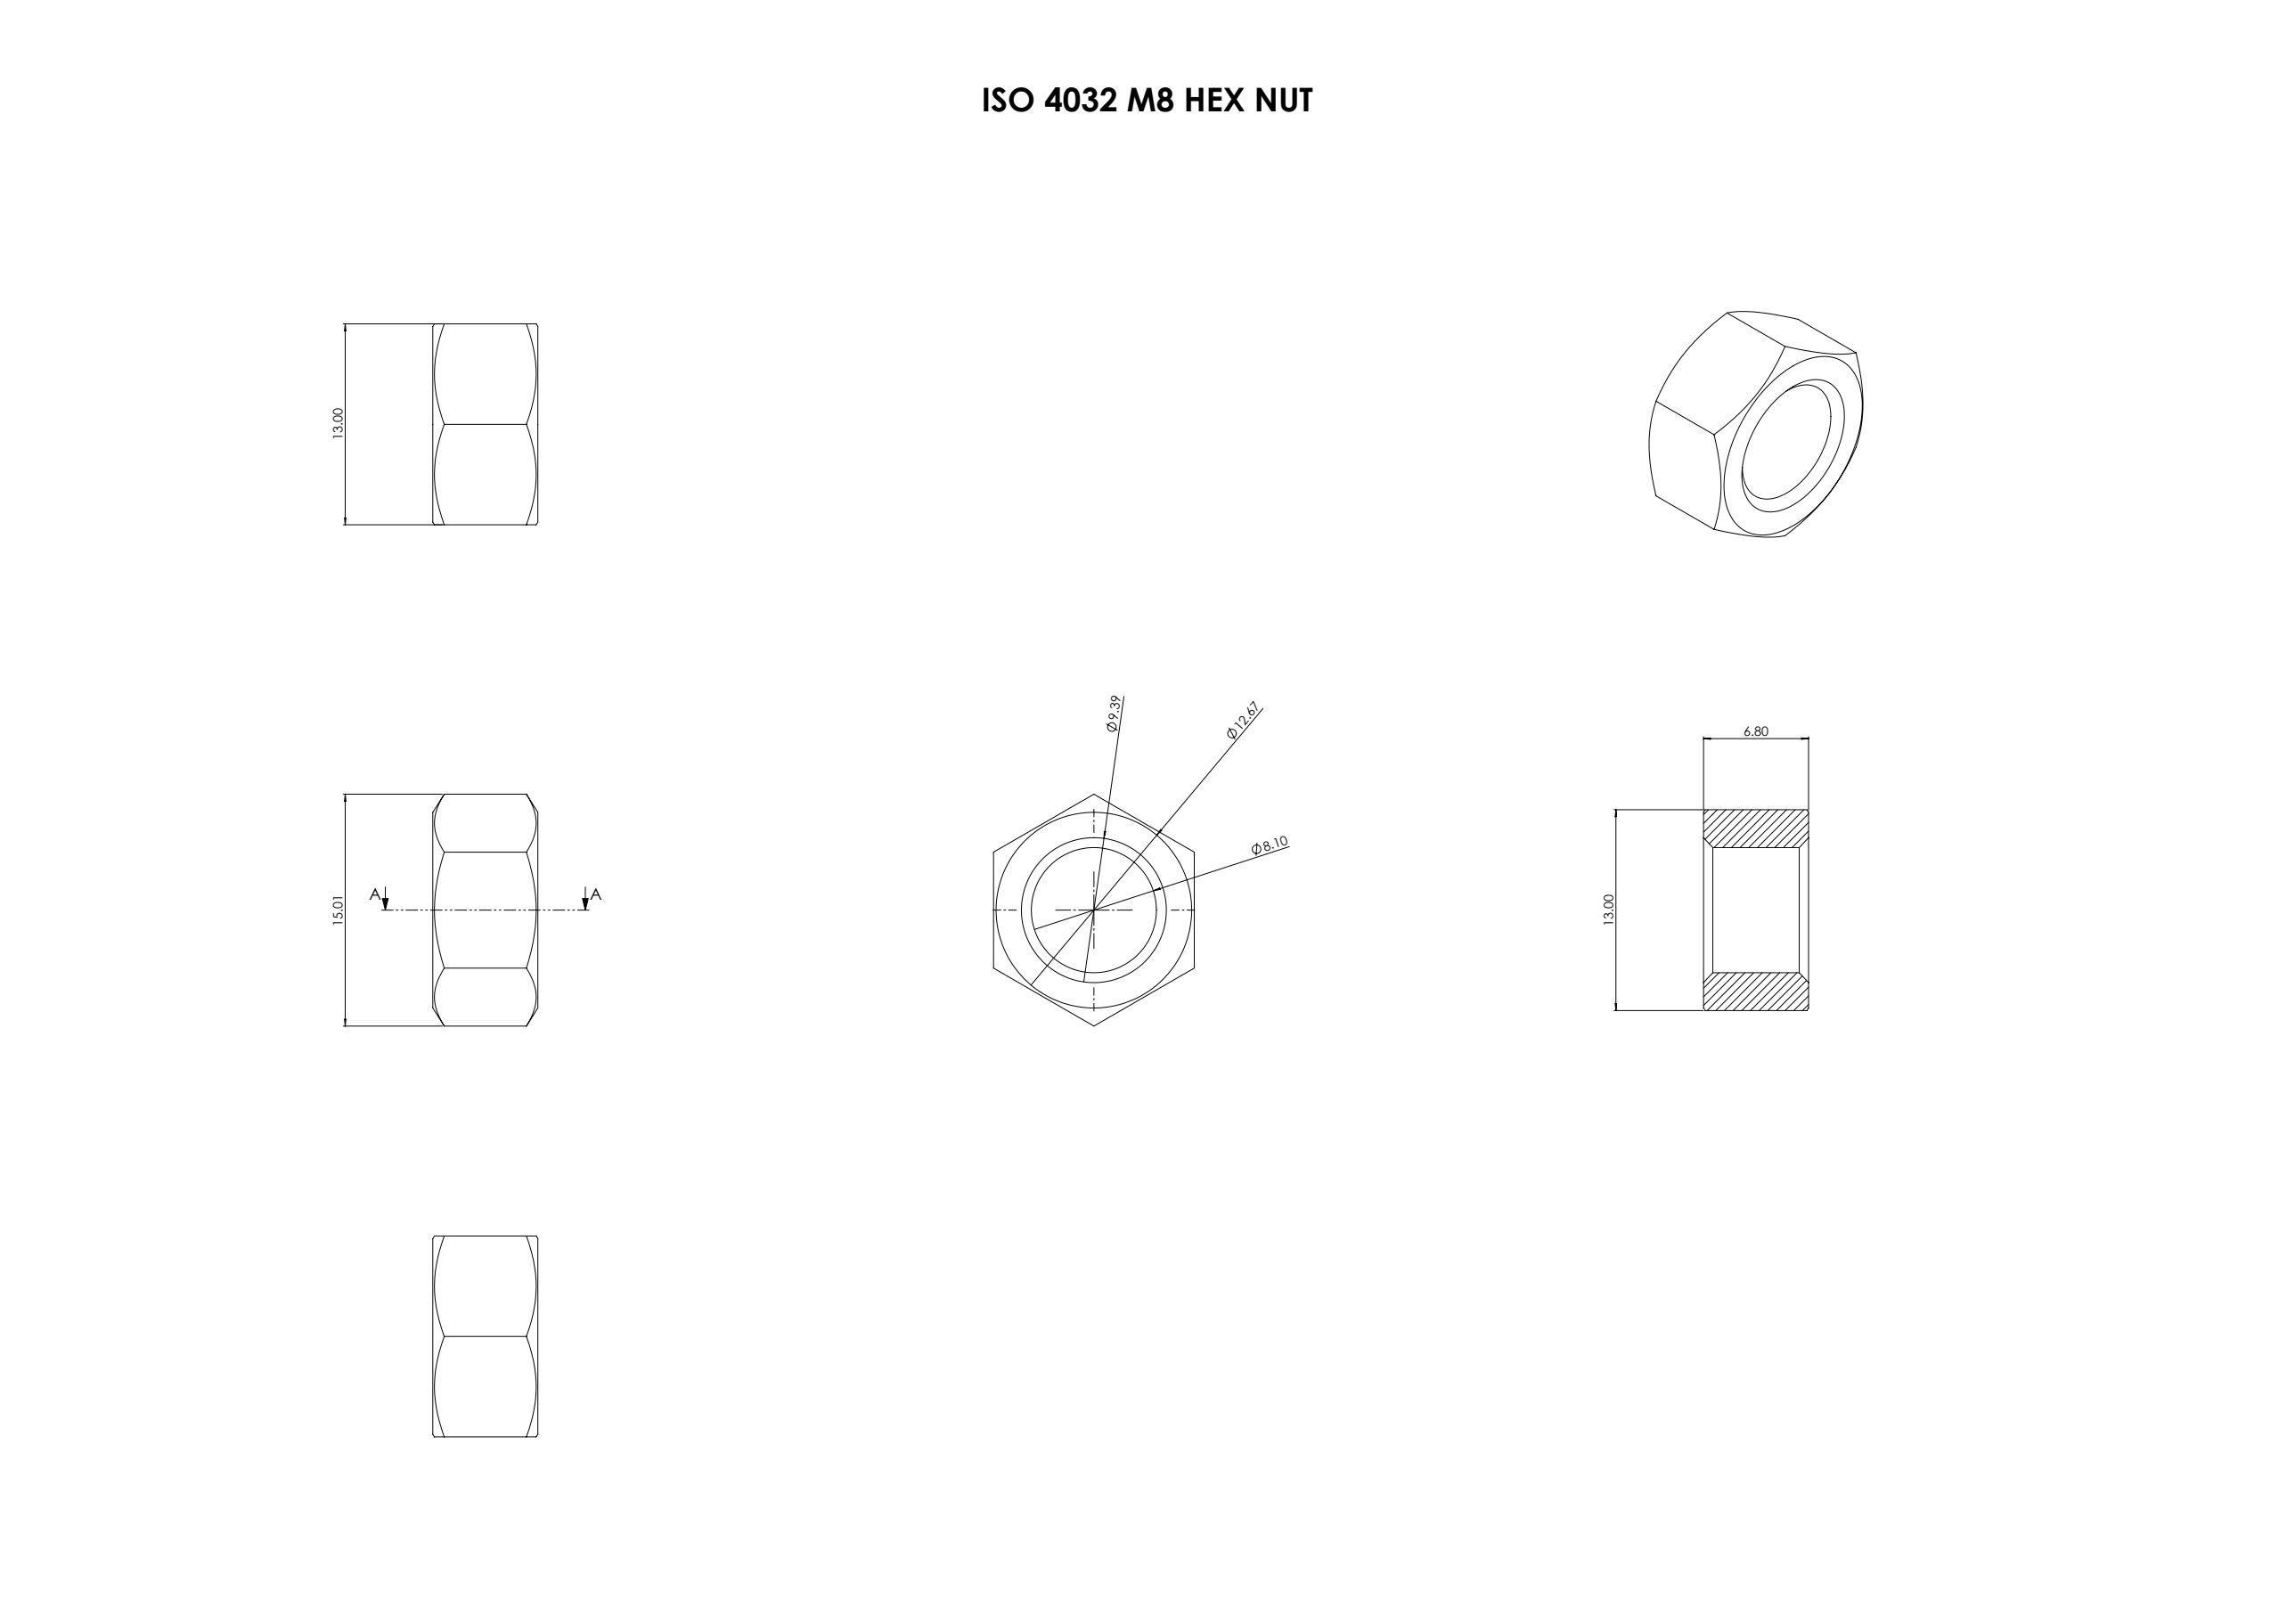
ISO-10303-21;
HEADER;
/* Generated by software containing ST-Developer
 * from STEP Tools, Inc. (www.steptools.com) 
 */

FILE_DESCRIPTION(
/* description */ (''),
/* implementation_level */ '2;1');

FILE_NAME(
/* name */ '14_ISO_4032_M8_Hex_Nut.step',
/* time_stamp */ '2026-10-11T08:27:52-07:00',
/* author */ (''),
/* organization */ (''),
/* preprocessor_version */ 'ST-DEVELOPER v20.2',
/* originating_system */ 'Autodesk Translation Framework v15.15.0.0',
/* authorisation */ '');

FILE_SCHEMA (('AUTOMOTIVE_DESIGN { 1 0 10303 214 3 1 1 }'));
ENDSEC;

DATA;
#10=MECHANICAL_DESIGN_GEOMETRIC_PRESENTATION_REPRESENTATION('',(#932),#94301);
#904=SHAPE_REPRESENTATION_RELATIONSHIP('SRR','None',#94384,#918);
#918=ADVANCED_BREP_SHAPE_REPRESENTATION('',(#946),#94300);
#932=STYLED_ITEM('',(#94588),#946);
#946=MANIFOLD_SOLID_BREP('Body1',#51031);
#1042=FACE_BOUND('',#18695,.T.);
#1043=FACE_BOUND('',#18697,.T.);
#1287=CYLINDRICAL_SURFACE('',#55318,4.05);
#6677=LINE('',#94156,#11205);
#6678=LINE('',#94160,#11206);
#6679=LINE('',#94164,#11207);
#6680=LINE('',#94170,#11208);
#6681=LINE('',#94196,#11209);
#6682=LINE('',#94201,#11210);
#6683=LINE('',#94204,#11211);
#6684=LINE('',#94210,#11212);
#6685=LINE('',#94224,#11213);
#6686=LINE('',#94230,#11214);
#6687=LINE('',#94232,#11215);
#11205=VECTOR('',#68145,4.425);
#11206=VECTOR('',#68150,4.05);
#11207=VECTOR('',#68155,4.425);
#11208=VECTOR('',#68162,7.09027674973257);
#11209=VECTOR('',#68165,10.);
#11210=VECTOR('',#68166,10.);
#11211=VECTOR('',#68169,10.);
#11212=VECTOR('',#68172,10.);
#11213=VECTOR('',#68175,7.09027674973257);
#11214=VECTOR('',#68180,10.);
#11215=VECTOR('',#68183,10.);
#13241=PLANE('',#55324);
#13242=PLANE('',#55325);
#13243=PLANE('',#55326);
#13244=PLANE('',#55329);
#13245=PLANE('',#55330);
#13246=PLANE('',#55331);
#13247=PLANE('',#55332);
#13248=PLANE('',#55333);
#15918=FACE_OUTER_BOUND('',#18683,.T.);
#15919=FACE_OUTER_BOUND('',#18684,.T.);
#15920=FACE_OUTER_BOUND('',#18685,.T.);
#15921=FACE_OUTER_BOUND('',#18686,.T.);
#15922=FACE_OUTER_BOUND('',#18687,.T.);
#15923=FACE_OUTER_BOUND('',#18688,.T.);
#15924=FACE_OUTER_BOUND('',#18689,.T.);
#15925=FACE_OUTER_BOUND('',#18690,.T.);
#15926=FACE_OUTER_BOUND('',#18691,.T.);
#15927=FACE_OUTER_BOUND('',#18692,.T.);
#15928=FACE_OUTER_BOUND('',#18693,.T.);
#15929=FACE_OUTER_BOUND('',#18694,.T.);
#15930=FACE_OUTER_BOUND('',#18696,.T.);
#18683=EDGE_LOOP('',(#48057,#48058,#48059,#48060));
#18684=EDGE_LOOP('',(#48061,#48062,#48063,#48064));
#18685=EDGE_LOOP('',(#48065,#48066,#48067,#48068));
#18686=EDGE_LOOP('',(#48069,#48070,#48071,#48072,#48073,#48074,#48075,#48076,
#48077));
#18687=EDGE_LOOP('',(#48078,#48079,#48080,#48081));
#18688=EDGE_LOOP('',(#48082,#48083,#48084,#48085));
#18689=EDGE_LOOP('',(#48086,#48087,#48088,#48089));
#18690=EDGE_LOOP('',(#48090,#48091,#48092,#48093,#48094,#48095,#48096,#48097,
#48098));
#18691=EDGE_LOOP('',(#48099,#48100,#48101,#48102));
#18692=EDGE_LOOP('',(#48103,#48104,#48105,#48106));
#18693=EDGE_LOOP('',(#48107,#48108,#48109,#48110));
#18694=EDGE_LOOP('',(#48111));
#18695=EDGE_LOOP('',(#48112));
#18696=EDGE_LOOP('',(#48113));
#18697=EDGE_LOOP('',(#48114));
#19562=(
BOUNDED_CURVE()
B_SPLINE_CURVE(2,(#94172,#94173,#94174),.UNSPECIFIED.,.F.,.F.)
B_SPLINE_CURVE_WITH_KNOTS((3,3),(0.0802593534055512,0.873558161927064),
 .UNSPECIFIED.)
CURVE()
GEOMETRIC_REPRESENTATION_ITEM()
RATIONAL_B_SPLINE_CURVE((1.03570012424137,1.19592349106096,1.03570012424137))
REPRESENTATION_ITEM('')
);
#19563=(
BOUNDED_CURVE()
B_SPLINE_CURVE(2,(#94176,#94177,#94178),.UNSPECIFIED.,.F.,.F.)
B_SPLINE_CURVE_WITH_KNOTS((3,3),(0.0802593534055512,0.873558161927064),
 .UNSPECIFIED.)
CURVE()
GEOMETRIC_REPRESENTATION_ITEM()
RATIONAL_B_SPLINE_CURVE((1.03570012424137,1.19592349106096,1.03570012424137))
REPRESENTATION_ITEM('')
);
#19564=(
BOUNDED_CURVE()
B_SPLINE_CURVE(2,(#94180,#94181,#94182),.UNSPECIFIED.,.F.,.F.)
B_SPLINE_CURVE_WITH_KNOTS((3,3),(0.0802593534055512,0.873558161927064),
 .UNSPECIFIED.)
CURVE()
GEOMETRIC_REPRESENTATION_ITEM()
RATIONAL_B_SPLINE_CURVE((1.03570012424137,1.19592349106096,1.03570012424137))
REPRESENTATION_ITEM('')
);
#19565=(
BOUNDED_CURVE()
B_SPLINE_CURVE(2,(#94184,#94185,#94186),.UNSPECIFIED.,.F.,.F.)
B_SPLINE_CURVE_WITH_KNOTS((3,3),(0.0802593534055512,0.873558161927064),
 .UNSPECIFIED.)
CURVE()
GEOMETRIC_REPRESENTATION_ITEM()
RATIONAL_B_SPLINE_CURVE((1.03570012424137,1.19592349106096,1.03570012424137))
REPRESENTATION_ITEM('')
);
#19566=(
BOUNDED_CURVE()
B_SPLINE_CURVE(2,(#94188,#94189,#94190),.UNSPECIFIED.,.F.,.F.)
B_SPLINE_CURVE_WITH_KNOTS((3,3),(0.0802593534055512,0.873558161927064),
 .UNSPECIFIED.)
CURVE()
GEOMETRIC_REPRESENTATION_ITEM()
RATIONAL_B_SPLINE_CURVE((1.03570012424137,1.19592349106096,1.03570012424137))
REPRESENTATION_ITEM('')
);
#19567=(
BOUNDED_CURVE()
B_SPLINE_CURVE(2,(#94191,#94192,#94193),.UNSPECIFIED.,.F.,.F.)
B_SPLINE_CURVE_WITH_KNOTS((3,3),(0.0802593534055513,0.873558161927064),
 .UNSPECIFIED.)
CURVE()
GEOMETRIC_REPRESENTATION_ITEM()
RATIONAL_B_SPLINE_CURVE((1.03570012424137,1.19592349106096,1.03570012424137))
REPRESENTATION_ITEM('')
);
#19568=(
BOUNDED_CURVE()
B_SPLINE_CURVE(2,(#94198,#94199,#94200),.UNSPECIFIED.,.F.,.F.)
B_SPLINE_CURVE_WITH_KNOTS((3,3),(0.080259353405551,0.873558161927064),
 .UNSPECIFIED.)
CURVE()
GEOMETRIC_REPRESENTATION_ITEM()
RATIONAL_B_SPLINE_CURVE((1.03570012424137,1.19592349106097,1.03570012424137))
REPRESENTATION_ITEM('')
);
#19569=(
BOUNDED_CURVE()
B_SPLINE_CURVE(2,(#94205,#94206,#94207),.UNSPECIFIED.,.F.,.F.)
B_SPLINE_CURVE_WITH_KNOTS((3,3),(0.0802593534055512,0.873558161927064),
 .UNSPECIFIED.)
CURVE()
GEOMETRIC_REPRESENTATION_ITEM()
RATIONAL_B_SPLINE_CURVE((1.03570012424137,1.19592349106096,1.03570012424137))
REPRESENTATION_ITEM('')
);
#19570=(
BOUNDED_CURVE()
B_SPLINE_CURVE(2,(#94211,#94212,#94213),.UNSPECIFIED.,.F.,.F.)
B_SPLINE_CURVE_WITH_KNOTS((3,3),(0.0802593534055513,0.873558161927064),
 .UNSPECIFIED.)
CURVE()
GEOMETRIC_REPRESENTATION_ITEM()
RATIONAL_B_SPLINE_CURVE((1.03570012424137,1.19592349106096,1.03570012424137))
REPRESENTATION_ITEM('')
);
#19571=(
BOUNDED_CURVE()
B_SPLINE_CURVE(2,(#94216,#94217,#94218),.UNSPECIFIED.,.F.,.F.)
B_SPLINE_CURVE_WITH_KNOTS((3,3),(0.0802593534055513,0.873558161927064),
 .UNSPECIFIED.)
CURVE()
GEOMETRIC_REPRESENTATION_ITEM()
RATIONAL_B_SPLINE_CURVE((1.03570012424137,1.19592349106096,1.03570012424137))
REPRESENTATION_ITEM('')
);
#19572=(
BOUNDED_CURVE()
B_SPLINE_CURVE(2,(#94220,#94221,#94222),.UNSPECIFIED.,.F.,.F.)
B_SPLINE_CURVE_WITH_KNOTS((3,3),(0.0802593534055512,0.873558161927064),
 .UNSPECIFIED.)
CURVE()
GEOMETRIC_REPRESENTATION_ITEM()
RATIONAL_B_SPLINE_CURVE((1.03570012424137,1.19592349106096,1.03570012424137))
REPRESENTATION_ITEM('')
);
#19573=(
BOUNDED_CURVE()
B_SPLINE_CURVE(2,(#94226,#94227,#94228),.UNSPECIFIED.,.F.,.F.)
B_SPLINE_CURVE_WITH_KNOTS((3,3),(0.0802593534055509,0.873558161927063),
 .UNSPECIFIED.)
CURVE()
GEOMETRIC_REPRESENTATION_ITEM()
RATIONAL_B_SPLINE_CURVE((1.03570012424137,1.19592349106096,1.03570012424137))
REPRESENTATION_ITEM('')
);
#20318=CIRCLE('',#55316,4.69285714285714);
#20319=CIRCLE('',#55317,4.05);
#20320=CIRCLE('',#55319,4.05);
#20321=CIRCLE('',#55321,4.69285714285714);
#20322=CIRCLE('',#55323,6.33323321723195);
#20323=CIRCLE('',#55328,6.33323321723195);
#25303=VERTEX_POINT('',#94153);
#25304=VERTEX_POINT('',#94155);
#25305=VERTEX_POINT('',#94159);
#25306=VERTEX_POINT('',#94163);
#25307=VERTEX_POINT('',#94167);
#25308=VERTEX_POINT('',#94169);
#25309=VERTEX_POINT('',#94171);
#25310=VERTEX_POINT('',#94175);
#25311=VERTEX_POINT('',#94179);
#25312=VERTEX_POINT('',#94183);
#25313=VERTEX_POINT('',#94187);
#25314=VERTEX_POINT('',#94195);
#25315=VERTEX_POINT('',#94197);
#25316=VERTEX_POINT('',#94203);
#25317=VERTEX_POINT('',#94209);
#25318=VERTEX_POINT('',#94215);
#25319=VERTEX_POINT('',#94219);
#25320=VERTEX_POINT('',#94223);
#32890=EDGE_CURVE('',#25303,#25303,#20318,.T.);
#32891=EDGE_CURVE('',#25303,#25304,#6677,.T.);
#32892=EDGE_CURVE('',#25304,#25304,#20319,.T.);
#32893=EDGE_CURVE('',#25304,#25305,#6678,.T.);
#32894=EDGE_CURVE('',#25305,#25305,#20320,.T.);
#32895=EDGE_CURVE('',#25305,#25306,#6679,.T.);
#32896=EDGE_CURVE('',#25306,#25306,#20321,.T.);
#32897=EDGE_CURVE('',#25307,#25307,#20322,.T.);
#32898=EDGE_CURVE('',#25307,#25308,#6680,.T.);
#32899=EDGE_CURVE('',#25309,#25308,#19562,.T.);
#32900=EDGE_CURVE('',#25310,#25309,#19563,.T.);
#32901=EDGE_CURVE('',#25311,#25310,#19564,.T.);
#32902=EDGE_CURVE('',#25312,#25311,#19565,.T.);
#32903=EDGE_CURVE('',#25313,#25312,#19566,.T.);
#32904=EDGE_CURVE('',#25308,#25313,#19567,.T.);
#32905=EDGE_CURVE('',#25312,#25314,#6681,.T.);
#32906=EDGE_CURVE('',#25314,#25315,#19568,.T.);
#32907=EDGE_CURVE('',#25313,#25315,#6682,.T.);
#32908=EDGE_CURVE('',#25311,#25316,#6683,.T.);
#32909=EDGE_CURVE('',#25316,#25314,#19569,.T.);
#32910=EDGE_CURVE('',#25310,#25317,#6684,.T.);
#32911=EDGE_CURVE('',#25317,#25316,#19570,.T.);
#32912=EDGE_CURVE('',#25318,#25317,#19571,.T.);
#32913=EDGE_CURVE('',#25319,#25318,#19572,.T.);
#32914=EDGE_CURVE('',#25319,#25320,#6685,.T.);
#32915=EDGE_CURVE('',#25320,#25320,#20323,.T.);
#32916=EDGE_CURVE('',#25315,#25319,#19573,.T.);
#32917=EDGE_CURVE('',#25309,#25318,#6686,.T.);
#32918=EDGE_CURVE('',#25308,#25319,#6687,.T.);
#48057=ORIENTED_EDGE('',*,*,#32890,.F.);
#48058=ORIENTED_EDGE('',*,*,#32891,.T.);
#48059=ORIENTED_EDGE('',*,*,#32892,.T.);
#48060=ORIENTED_EDGE('',*,*,#32891,.F.);
#48061=ORIENTED_EDGE('',*,*,#32892,.F.);
#48062=ORIENTED_EDGE('',*,*,#32893,.T.);
#48063=ORIENTED_EDGE('',*,*,#32894,.T.);
#48064=ORIENTED_EDGE('',*,*,#32893,.F.);
#48065=ORIENTED_EDGE('',*,*,#32894,.F.);
#48066=ORIENTED_EDGE('',*,*,#32895,.T.);
#48067=ORIENTED_EDGE('',*,*,#32896,.F.);
#48068=ORIENTED_EDGE('',*,*,#32895,.F.);
#48069=ORIENTED_EDGE('',*,*,#32897,.F.);
#48070=ORIENTED_EDGE('',*,*,#32898,.T.);
#48071=ORIENTED_EDGE('',*,*,#32899,.F.);
#48072=ORIENTED_EDGE('',*,*,#32900,.F.);
#48073=ORIENTED_EDGE('',*,*,#32901,.F.);
#48074=ORIENTED_EDGE('',*,*,#32902,.F.);
#48075=ORIENTED_EDGE('',*,*,#32903,.F.);
#48076=ORIENTED_EDGE('',*,*,#32904,.F.);
#48077=ORIENTED_EDGE('',*,*,#32898,.F.);
#48078=ORIENTED_EDGE('',*,*,#32903,.T.);
#48079=ORIENTED_EDGE('',*,*,#32905,.T.);
#48080=ORIENTED_EDGE('',*,*,#32906,.T.);
#48081=ORIENTED_EDGE('',*,*,#32907,.F.);
#48082=ORIENTED_EDGE('',*,*,#32902,.T.);
#48083=ORIENTED_EDGE('',*,*,#32908,.T.);
#48084=ORIENTED_EDGE('',*,*,#32909,.T.);
#48085=ORIENTED_EDGE('',*,*,#32905,.F.);
#48086=ORIENTED_EDGE('',*,*,#32901,.T.);
#48087=ORIENTED_EDGE('',*,*,#32910,.T.);
#48088=ORIENTED_EDGE('',*,*,#32911,.T.);
#48089=ORIENTED_EDGE('',*,*,#32908,.F.);
#48090=ORIENTED_EDGE('',*,*,#32906,.F.);
#48091=ORIENTED_EDGE('',*,*,#32909,.F.);
#48092=ORIENTED_EDGE('',*,*,#32911,.F.);
#48093=ORIENTED_EDGE('',*,*,#32912,.F.);
#48094=ORIENTED_EDGE('',*,*,#32913,.F.);
#48095=ORIENTED_EDGE('',*,*,#32914,.T.);
#48096=ORIENTED_EDGE('',*,*,#32915,.F.);
#48097=ORIENTED_EDGE('',*,*,#32914,.F.);
#48098=ORIENTED_EDGE('',*,*,#32916,.F.);
#48099=ORIENTED_EDGE('',*,*,#32900,.T.);
#48100=ORIENTED_EDGE('',*,*,#32917,.T.);
#48101=ORIENTED_EDGE('',*,*,#32912,.T.);
#48102=ORIENTED_EDGE('',*,*,#32910,.F.);
#48103=ORIENTED_EDGE('',*,*,#32904,.T.);
#48104=ORIENTED_EDGE('',*,*,#32907,.T.);
#48105=ORIENTED_EDGE('',*,*,#32916,.T.);
#48106=ORIENTED_EDGE('',*,*,#32918,.F.);
#48107=ORIENTED_EDGE('',*,*,#32899,.T.);
#48108=ORIENTED_EDGE('',*,*,#32918,.T.);
#48109=ORIENTED_EDGE('',*,*,#32913,.T.);
#48110=ORIENTED_EDGE('',*,*,#32917,.F.);
#48111=ORIENTED_EDGE('',*,*,#32915,.T.);
#48112=ORIENTED_EDGE('',*,*,#32896,.T.);
#48113=ORIENTED_EDGE('',*,*,#32897,.T.);
#48114=ORIENTED_EDGE('',*,*,#32890,.T.);
#48332=CONICAL_SURFACE('',#55315,4.425,0.819867264396957);
#48333=CONICAL_SURFACE('',#55320,4.425,0.819867264396957);
#48334=CONICAL_SURFACE('',#55322,7.09027674973257,1.0071944566367);
#48335=CONICAL_SURFACE('',#55327,7.09027674973257,1.0071944566367);
#51005=ADVANCED_FACE('',(#15918),#48332,.F.);
#51006=ADVANCED_FACE('',(#15919),#1287,.F.);
#51007=ADVANCED_FACE('',(#15920),#48333,.F.);
#51008=ADVANCED_FACE('',(#15921),#48334,.T.);
#51009=ADVANCED_FACE('',(#15922),#13241,.T.);
#51010=ADVANCED_FACE('',(#15923),#13242,.T.);
#51011=ADVANCED_FACE('',(#15924),#13243,.T.);
#51012=ADVANCED_FACE('',(#15925),#48335,.T.);
#51013=ADVANCED_FACE('',(#15926),#13244,.T.);
#51014=ADVANCED_FACE('',(#15927),#13245,.T.);
#51015=ADVANCED_FACE('',(#15928),#13246,.T.);
#51016=ADVANCED_FACE('',(#15929,#1042),#13247,.T.);
#51017=ADVANCED_FACE('',(#15930,#1043),#13248,.F.);
#51031=CLOSED_SHELL('',(#51005,#51006,#51007,#51008,#51009,#51010,#51011,
#51012,#51013,#51014,#51015,#51016,#51017));
#55314=AXIS2_PLACEMENT_3D('',#94151,#68139,#68140);
#55315=AXIS2_PLACEMENT_3D('',#94152,#68141,#68142);
#55316=AXIS2_PLACEMENT_3D('',#94154,#68143,#68144);
#55317=AXIS2_PLACEMENT_3D('',#94157,#68146,#68147);
#55318=AXIS2_PLACEMENT_3D('',#94158,#68148,#68149);
#55319=AXIS2_PLACEMENT_3D('',#94161,#68151,#68152);
#55320=AXIS2_PLACEMENT_3D('',#94162,#68153,#68154);
#55321=AXIS2_PLACEMENT_3D('',#94165,#68156,#68157);
#55322=AXIS2_PLACEMENT_3D('',#94166,#68158,#68159);
#55323=AXIS2_PLACEMENT_3D('',#94168,#68160,#68161);
#55324=AXIS2_PLACEMENT_3D('',#94194,#68163,#68164);
#55325=AXIS2_PLACEMENT_3D('',#94202,#68167,#68168);
#55326=AXIS2_PLACEMENT_3D('',#94208,#68170,#68171);
#55327=AXIS2_PLACEMENT_3D('',#94214,#68173,#68174);
#55328=AXIS2_PLACEMENT_3D('',#94225,#68176,#68177);
#55329=AXIS2_PLACEMENT_3D('',#94229,#68178,#68179);
#55330=AXIS2_PLACEMENT_3D('',#94231,#68181,#68182);
#55331=AXIS2_PLACEMENT_3D('',#94233,#68184,#68185);
#55332=AXIS2_PLACEMENT_3D('',#94234,#68186,#68187);
#55333=AXIS2_PLACEMENT_3D('',#94235,#68188,#68189);
#68139=DIRECTION('axis',(0.,0.,1.));
#68140=DIRECTION('refdir',(1.,0.,0.));
#68141=DIRECTION('center_axis',(-1.,0.,0.));
#68142=DIRECTION('ref_axis',(0.,1.,0.));
#68143=DIRECTION('center_axis',(1.,0.,0.));
#68144=DIRECTION('ref_axis',(0.,1.,0.));
#68145=DIRECTION('',(0.682318250360011,0.731055268242869,8.95284494253439E-17));
#68146=DIRECTION('center_axis',(1.,0.,0.));
#68147=DIRECTION('ref_axis',(0.,0.,-1.));
#68148=DIRECTION('center_axis',(1.,0.,0.));
#68149=DIRECTION('ref_axis',(0.,1.,0.));
#68150=DIRECTION('',(1.,0.,0.));
#68151=DIRECTION('center_axis',(1.,0.,0.));
#68152=DIRECTION('ref_axis',(0.,0.,-1.));
#68153=DIRECTION('center_axis',(1.,0.,0.));
#68154=DIRECTION('ref_axis',(0.,1.,0.));
#68155=DIRECTION('',(0.682318250360011,-0.731055268242869,-8.9528449425344E-17));
#68156=DIRECTION('center_axis',(-1.,0.,0.));
#68157=DIRECTION('ref_axis',(0.,1.,0.));
#68158=DIRECTION('center_axis',(1.,0.,0.));
#68159=DIRECTION('ref_axis',(0.,1.,0.));
#68160=DIRECTION('center_axis',(-1.,0.,0.));
#68161=DIRECTION('ref_axis',(0.,1.,0.));
#68162=DIRECTION('',(0.534234448563085,-0.845336355522756,-1.03523846199383E-16));
#68163=DIRECTION('center_axis',(0.,-2.95840413289779E-16,-1.));
#68164=DIRECTION('ref_axis',(0.,1.,-2.95840413289779E-16));
#68165=DIRECTION('',(1.,0.,0.));
#68166=DIRECTION('',(1.,0.,0.));
#68167=DIRECTION('center_axis',(0.,0.866025403784439,-0.5));
#68168=DIRECTION('ref_axis',(0.,0.5,0.866025403784439));
#68169=DIRECTION('',(1.,0.,0.));
#68170=DIRECTION('center_axis',(0.,0.866025403784439,0.5));
#68171=DIRECTION('ref_axis',(0.,-0.5,0.866025403784439));
#68172=DIRECTION('',(1.,0.,0.));
#68173=DIRECTION('center_axis',(-1.,0.,0.));
#68174=DIRECTION('ref_axis',(0.,1.,0.));
#68175=DIRECTION('',(0.534234448563085,0.845336355522756,1.03523846199383E-16));
#68176=DIRECTION('center_axis',(1.,0.,0.));
#68177=DIRECTION('ref_axis',(0.,1.,0.));
#68178=DIRECTION('center_axis',(0.,1.4792020664489E-16,1.));
#68179=DIRECTION('ref_axis',(0.,-1.,1.4792020664489E-16));
#68180=DIRECTION('',(1.,0.,0.));
#68181=DIRECTION('center_axis',(0.,-0.866025403784439,-0.5));
#68182=DIRECTION('ref_axis',(0.,0.5,-0.866025403784439));
#68183=DIRECTION('',(1.,0.,0.));
#68184=DIRECTION('center_axis',(0.,-0.866025403784439,0.5));
#68185=DIRECTION('ref_axis',(0.,-0.5,-0.866025403784439));
#68186=DIRECTION('center_axis',(1.,0.,0.));
#68187=DIRECTION('ref_axis',(0.,0.,-1.));
#68188=DIRECTION('center_axis',(1.,0.,0.));
#68189=DIRECTION('ref_axis',(0.,0.,-1.));
#94151=CARTESIAN_POINT('',(0.,0.,0.));
#94152=CARTESIAN_POINT('Origin',(0.25,0.,0.));
#94153=CARTESIAN_POINT('',(0.,-4.69285714285714,-5.74709247885579E-16));
#94154=CARTESIAN_POINT('Origin',(0.,0.,0.));
#94155=CARTESIAN_POINT('',(0.600000000000001,-4.05,-4.95981953654678E-16));
#94156=CARTESIAN_POINT('',(0.25,-4.425,-5.41906208622704E-16));
#94157=CARTESIAN_POINT('Origin',(0.600000000000001,0.,0.));
#94158=CARTESIAN_POINT('Origin',(3.4,0.,0.));
#94159=CARTESIAN_POINT('',(6.2,-4.05,-4.95981953654678E-16));
#94160=CARTESIAN_POINT('',(3.4,-4.05,-4.95981953654678E-16));
#94161=CARTESIAN_POINT('Origin',(6.2,0.,0.));
#94162=CARTESIAN_POINT('Origin',(6.55,0.,0.));
#94163=CARTESIAN_POINT('',(6.8,-4.69285714285714,5.74709247885579E-16));
#94164=CARTESIAN_POINT('',(6.55,-4.425,-5.41906208622704E-16));
#94165=CARTESIAN_POINT('Origin',(6.8,0.,0.));
#94166=CARTESIAN_POINT('Origin',(0.478435277841104,0.,0.));
#94167=CARTESIAN_POINT('',(0.,-6.33323321723195,7.75597378773681E-16));
#94168=CARTESIAN_POINT('Origin',(0.,0.,0.));
#94169=CARTESIAN_POINT('',(0.740881278116643,-7.50555349946513,9.19165206894919E-16));
#94170=CARTESIAN_POINT('',(0.478435277841104,-7.09027674973257,-8.68308472662889E-16));
#94171=CARTESIAN_POINT('',(0.740881278116643,-3.75277674973257,6.5));
#94172=CARTESIAN_POINT('Ctrl Pts',(0.740881278116643,-3.75277674973257,
6.5));
#94173=CARTESIAN_POINT('Ctrl Pts',(-0.444955935896173,-5.62916512459885,
3.25));
#94174=CARTESIAN_POINT('Ctrl Pts',(0.740881278116643,-7.50555349946513,
9.19165206894919E-16));
#94175=CARTESIAN_POINT('',(0.740881278116644,3.75277674973257,6.5));
#94176=CARTESIAN_POINT('Ctrl Pts',(0.740881278116644,3.75277674973257,6.5));
#94177=CARTESIAN_POINT('Ctrl Pts',(-0.444955935896173,-5.55111512312578E-15,
6.5));
#94178=CARTESIAN_POINT('Ctrl Pts',(0.740881278116643,-3.75277674973257,
6.5));
#94179=CARTESIAN_POINT('',(0.740881278116643,7.50555349946513,0.));
#94180=CARTESIAN_POINT('Ctrl Pts',(0.740881278116643,7.50555349946513,0.));
#94181=CARTESIAN_POINT('Ctrl Pts',(-0.444955935896173,5.62916512459885,
3.25000000000001));
#94182=CARTESIAN_POINT('Ctrl Pts',(0.740881278116644,3.75277674973257,6.5));
#94183=CARTESIAN_POINT('',(0.740881278116644,3.75277674973257,-6.5));
#94184=CARTESIAN_POINT('Ctrl Pts',(0.740881278116644,3.75277674973257,-6.5));
#94185=CARTESIAN_POINT('Ctrl Pts',(-0.444955935896173,5.62916512459886,
-3.24999999999999));
#94186=CARTESIAN_POINT('Ctrl Pts',(0.740881278116643,7.50555349946513,0.));
#94187=CARTESIAN_POINT('',(0.740881278116643,-3.75277674973257,-6.5));
#94188=CARTESIAN_POINT('Ctrl Pts',(0.740881278116643,-3.75277674973257,
-6.5));
#94189=CARTESIAN_POINT('Ctrl Pts',(-0.444955935896175,4.44089209850063E-15,
-6.5));
#94190=CARTESIAN_POINT('Ctrl Pts',(0.740881278116644,3.75277674973257,-6.5));
#94191=CARTESIAN_POINT('Ctrl Pts',(0.740881278116643,-7.50555349946513,
9.19165206894919E-16));
#94192=CARTESIAN_POINT('Ctrl Pts',(-0.444955935896174,-5.62916512459885,
-3.25));
#94193=CARTESIAN_POINT('Ctrl Pts',(0.740881278116643,-3.75277674973257,
-6.5));
#94194=CARTESIAN_POINT('Origin',(0.,-3.75277674973257,-6.5));
#94195=CARTESIAN_POINT('',(6.05911872188336,3.75277674973257,-6.5));
#94196=CARTESIAN_POINT('',(0.,3.75277674973257,-6.5));
#94197=CARTESIAN_POINT('',(6.05911872188336,-3.75277674973257,-6.5));
#94198=CARTESIAN_POINT('Ctrl Pts',(6.05911872188336,3.75277674973257,-6.5));
#94199=CARTESIAN_POINT('Ctrl Pts',(7.24495593589617,-9.99200722162641E-15,
-6.5));
#94200=CARTESIAN_POINT('Ctrl Pts',(6.05911872188336,-3.75277674973257,-6.5));
#94201=CARTESIAN_POINT('',(0.,-3.75277674973257,-6.5));
#94202=CARTESIAN_POINT('Origin',(0.,3.75277674973257,-6.5));
#94203=CARTESIAN_POINT('',(6.05911872188336,7.50555349946513,0.));
#94204=CARTESIAN_POINT('',(0.,7.50555349946513,0.));
#94205=CARTESIAN_POINT('Ctrl Pts',(6.05911872188336,7.50555349946513,0.));
#94206=CARTESIAN_POINT('Ctrl Pts',(7.24495593589617,5.62916512459885,-3.25000000000001));
#94207=CARTESIAN_POINT('Ctrl Pts',(6.05911872188336,3.75277674973257,-6.5));
#94208=CARTESIAN_POINT('Origin',(0.,7.50555349946513,0.));
#94209=CARTESIAN_POINT('',(6.05911872188336,3.75277674973257,6.5));
#94210=CARTESIAN_POINT('',(0.,3.75277674973257,6.5));
#94211=CARTESIAN_POINT('Ctrl Pts',(6.05911872188336,3.75277674973257,6.5));
#94212=CARTESIAN_POINT('Ctrl Pts',(7.24495593589617,5.62916512459885,3.25));
#94213=CARTESIAN_POINT('Ctrl Pts',(6.05911872188336,7.50555349946513,0.));
#94214=CARTESIAN_POINT('Origin',(6.3215647221589,0.,0.));
#94215=CARTESIAN_POINT('',(6.05911872188336,-3.75277674973257,6.5));
#94216=CARTESIAN_POINT('Ctrl Pts',(6.05911872188336,-3.75277674973257,6.5));
#94217=CARTESIAN_POINT('Ctrl Pts',(7.24495593589618,7.7715611723761E-15,
6.5));
#94218=CARTESIAN_POINT('Ctrl Pts',(6.05911872188336,3.75277674973257,6.5));
#94219=CARTESIAN_POINT('',(6.05911872188336,-7.50555349946513,9.19165206894919E-16));
#94220=CARTESIAN_POINT('Ctrl Pts',(6.05911872188336,-7.50555349946513,9.19165206894919E-16));
#94221=CARTESIAN_POINT('Ctrl Pts',(7.24495593589617,-5.62916512459885,3.25000000000001));
#94222=CARTESIAN_POINT('Ctrl Pts',(6.05911872188336,-3.75277674973257,6.5));
#94223=CARTESIAN_POINT('',(6.8,-6.33323321723195,-7.75597378773681E-16));
#94224=CARTESIAN_POINT('',(6.3215647221589,-7.09027674973257,-8.68308472662889E-16));
#94225=CARTESIAN_POINT('Origin',(6.8,0.,0.));
#94226=CARTESIAN_POINT('Ctrl Pts',(6.05911872188336,-3.75277674973257,-6.5));
#94227=CARTESIAN_POINT('Ctrl Pts',(7.24495593589618,-5.62916512459886,-3.24999999999999));
#94228=CARTESIAN_POINT('Ctrl Pts',(6.05911872188336,-7.50555349946513,9.19165206894919E-16));
#94229=CARTESIAN_POINT('Origin',(0.,3.75277674973257,6.5));
#94230=CARTESIAN_POINT('',(0.,-3.75277674973257,6.5));
#94231=CARTESIAN_POINT('Origin',(0.,-7.50555349946513,9.19165206894919E-16));
#94232=CARTESIAN_POINT('',(0.,-7.50555349946513,9.19165206894919E-16));
#94233=CARTESIAN_POINT('Origin',(0.,-3.75277674973257,6.5));
#94234=CARTESIAN_POINT('Origin',(6.8,0.,0.));
#94235=CARTESIAN_POINT('Origin',(0.,0.,0.));
#94284=UNCERTAINTY_MEASURE_WITH_UNIT(LENGTH_MEASURE(0.01),#94302,
'DISTANCE_ACCURACY_VALUE',
'Maximum model space distance between geometric entities at asserted c
onnectivities');
#94285=UNCERTAINTY_MEASURE_WITH_UNIT(LENGTH_MEASURE(0.01),#94302,
'DISTANCE_ACCURACY_VALUE',
'Maximum model space distance between geometric entities at asserted c
onnectivities');
#94300=(
GEOMETRIC_REPRESENTATION_CONTEXT(3)
GLOBAL_UNCERTAINTY_ASSIGNED_CONTEXT((#94284))
GLOBAL_UNIT_ASSIGNED_CONTEXT((#94302,#94304,#94305))
REPRESENTATION_CONTEXT('','3D')
);
#94301=(
GEOMETRIC_REPRESENTATION_CONTEXT(3)
GLOBAL_UNCERTAINTY_ASSIGNED_CONTEXT((#94285))
GLOBAL_UNIT_ASSIGNED_CONTEXT((#94302,#94304,#94305))
REPRESENTATION_CONTEXT('','3D')
);
#94302=(
LENGTH_UNIT()
NAMED_UNIT(*)
SI_UNIT(.MILLI.,.METRE.)
);
#94304=(
NAMED_UNIT(*)
PLANE_ANGLE_UNIT()
SI_UNIT($,.RADIAN.)
);
#94305=(
NAMED_UNIT(*)
SI_UNIT($,.STERADIAN.)
SOLID_ANGLE_UNIT()
);
#94320=SHAPE_DEFINITION_REPRESENTATION(#94335,#94384);
#94335=PRODUCT_DEFINITION_SHAPE('',$,#94400);
#94384=SHAPE_REPRESENTATION('',(#55314),#94300);
#94385=PRODUCT_DEFINITION_CONTEXT('part definition',#94432,'design');
#94400=PRODUCT_DEFINITION('2026-10-11-08-26-51-541',
'14_ISO_4032_M8_Hex_Nut',#94415,#94385);
#94415=PRODUCT_DEFINITION_FORMATION('',$,#94448);
#94432=APPLICATION_CONTEXT(
'Core Data for Automotive Mechanical Design Process');
#94433=PRODUCT_CONTEXT('part definition',#94432,'mechanical');
#94448=PRODUCT('2026-10-11-08-26-51-541','14_ISO_4032_M8_Hex_Nut',$,(#94433));
#94582=COLOUR_RGB('Black',0.12,0.14,0.17);
#94583=FILL_AREA_STYLE_COLOUR('',#94582);
#94584=FILL_AREA_STYLE('',(#94583));
#94585=SURFACE_STYLE_FILL_AREA(#94584);
#94586=SURFACE_SIDE_STYLE('',(#94585));
#94587=SURFACE_STYLE_USAGE(.BOTH.,#94586);
#94588=PRESENTATION_STYLE_ASSIGNMENT((#94587));
ENDSEC;
END-ISO-10303-21;
